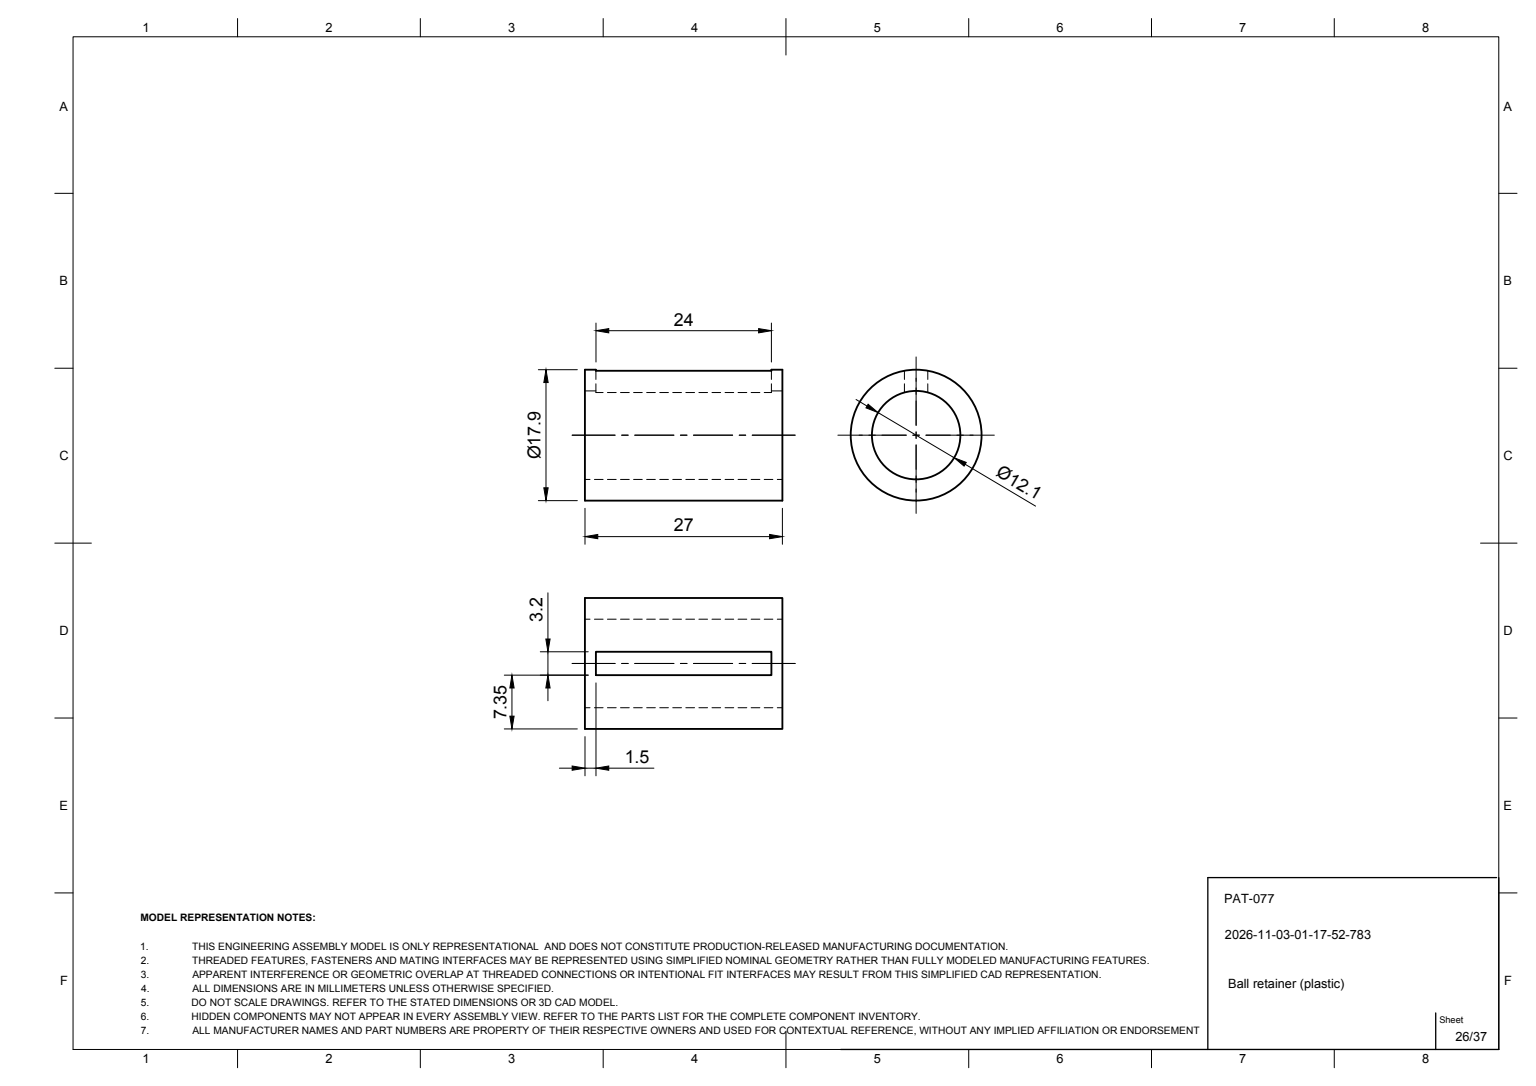
ISO-10303-21;
HEADER;
/* Generated by software containing ST-Developer
 * from STEP Tools, Inc. (www.steptools.com) 
 */

FILE_DESCRIPTION(
/* description */ ('Pallet stop with pneumatic fitting'),
/* implementation_level */ '2;1');

FILE_NAME(
/* name */ 'Ball retainer (plastic).step',
/* time_stamp */ '2026-10-27T10:51:41-07:00',
/* author */ (''),
/* organization */ (''),
/* preprocessor_version */ 'ST-DEVELOPER v20.2',
/* originating_system */ 'Autodesk Translation Framework v15.17.0.0',
/* authorisation */ '');

FILE_SCHEMA (('AUTOMOTIVE_DESIGN { 1 0 10303 214 3 1 1 }'));
ENDSEC;

DATA;
#10=MECHANICAL_DESIGN_GEOMETRIC_PRESENTATION_REPRESENTATION('',(#376),#10265);
#312=SHAPE_REPRESENTATION_RELATIONSHIP('SRR','None',#10426,#344);
#344=ADVANCED_BREP_SHAPE_REPRESENTATION('',(#408),#10250);
#376=STYLED_ITEM('',(#10648),#408);
#408=MANIFOLD_SOLID_BREP('Body1',#5064);
#511=FACE_BOUND('',#1322,.T.);
#512=FACE_BOUND('',#1324,.T.);
#513=FACE_BOUND('',#1326,.T.);
#514=FACE_BOUND('',#1328,.T.);
#643=PLANE('',#5785);
#644=PLANE('',#5788);
#645=PLANE('',#5789);
#646=PLANE('',#5792);
#647=PLANE('',#5793);
#648=PLANE('',#5798);
#911=FACE_OUTER_BOUND('',#1317,.T.);
#912=FACE_OUTER_BOUND('',#1318,.T.);
#913=FACE_OUTER_BOUND('',#1319,.T.);
#914=FACE_OUTER_BOUND('',#1320,.T.);
#915=FACE_OUTER_BOUND('',#1321,.T.);
#916=FACE_OUTER_BOUND('',#1323,.T.);
#917=FACE_OUTER_BOUND('',#1325,.T.);
#918=FACE_OUTER_BOUND('',#1327,.T.);
#1317=EDGE_LOOP('',(#4060,#4061,#4062,#4063));
#1318=EDGE_LOOP('',(#4064,#4065,#4066,#4067));
#1319=EDGE_LOOP('',(#4068,#4069,#4070,#4071));
#1320=EDGE_LOOP('',(#4072,#4073,#4074,#4075));
#1321=EDGE_LOOP('',(#4076));
#1322=EDGE_LOOP('',(#4077));
#1323=EDGE_LOOP('',(#4078,#4079,#4080,#4081));
#1324=EDGE_LOOP('',(#4082,#4083,#4084,#4085));
#1325=EDGE_LOOP('',(#4086));
#1326=EDGE_LOOP('',(#4087));
#1327=EDGE_LOOP('',(#4088,#4089,#4090,#4091));
#1328=EDGE_LOOP('',(#4092,#4093,#4094,#4095));
#1652=LINE('',#9434,#1987);
#1653=LINE('',#9437,#1988);
#1654=LINE('',#9440,#1989);
#1655=LINE('',#9442,#1990);
#1656=LINE('',#9443,#1991);
#1657=LINE('',#9449,#1992);
#1658=LINE('',#9451,#1993);
#1659=LINE('',#9452,#1994);
#1660=LINE('',#9461,#1995);
#1661=LINE('',#9466,#1996);
#1987=VECTOR('',#6961,1.);
#1988=VECTOR('',#6964,1.);
#1989=VECTOR('',#6967,1.);
#1990=VECTOR('',#6968,1.);
#1991=VECTOR('',#6969,1.);
#1992=VECTOR('',#6976,1.);
#1993=VECTOR('',#6979,1.);
#1994=VECTOR('',#6980,1.);
#1995=VECTOR('',#6991,0.895);
#1996=VECTOR('',#6998,0.605);
#2316=CIRCLE('',#5786,0.895);
#2317=CIRCLE('',#5787,0.605);
#2318=CIRCLE('',#5790,0.895);
#2319=CIRCLE('',#5791,0.605);
#2320=CIRCLE('',#5794,0.895);
#2321=CIRCLE('',#5795,0.605);
#2322=CIRCLE('',#5797,0.895);
#2323=CIRCLE('',#5799,0.605);
#2622=VERTEX_POINT('',#9430);
#2623=VERTEX_POINT('',#9431);
#2624=VERTEX_POINT('',#9433);
#2625=VERTEX_POINT('',#9435);
#2626=VERTEX_POINT('',#9439);
#2627=VERTEX_POINT('',#9441);
#2628=VERTEX_POINT('',#9445);
#2629=VERTEX_POINT('',#9447);
#2630=VERTEX_POINT('',#9454);
#2631=VERTEX_POINT('',#9456);
#2632=VERTEX_POINT('',#9459);
#2633=VERTEX_POINT('',#9463);
#3129=EDGE_CURVE('',#2622,#2623,#2316,.T.);
#3130=EDGE_CURVE('',#2624,#2622,#1652,.T.);
#3131=EDGE_CURVE('',#2625,#2624,#2317,.T.);
#3132=EDGE_CURVE('',#2623,#2625,#1653,.T.);
#3133=EDGE_CURVE('',#2623,#2626,#1654,.T.);
#3134=EDGE_CURVE('',#2627,#2625,#1655,.T.);
#3135=EDGE_CURVE('',#2627,#2626,#1656,.T.);
#3136=EDGE_CURVE('',#2626,#2628,#2318,.T.);
#3137=EDGE_CURVE('',#2629,#2627,#2319,.T.);
#3138=EDGE_CURVE('',#2628,#2629,#1657,.T.);
#3139=EDGE_CURVE('',#2628,#2622,#1658,.T.);
#3140=EDGE_CURVE('',#2624,#2629,#1659,.T.);
#3141=EDGE_CURVE('',#2630,#2630,#2320,.T.);
#3142=EDGE_CURVE('',#2631,#2631,#2321,.T.);
#3143=EDGE_CURVE('',#2632,#2632,#2322,.T.);
#3144=EDGE_CURVE('',#2632,#2630,#1660,.T.);
#3145=EDGE_CURVE('',#2633,#2633,#2323,.T.);
#3146=EDGE_CURVE('',#2633,#2631,#1661,.T.);
#4060=ORIENTED_EDGE('',*,*,#3129,.F.);
#4061=ORIENTED_EDGE('',*,*,#3130,.F.);
#4062=ORIENTED_EDGE('',*,*,#3131,.F.);
#4063=ORIENTED_EDGE('',*,*,#3132,.F.);
#4064=ORIENTED_EDGE('',*,*,#3133,.F.);
#4065=ORIENTED_EDGE('',*,*,#3132,.T.);
#4066=ORIENTED_EDGE('',*,*,#3134,.F.);
#4067=ORIENTED_EDGE('',*,*,#3135,.T.);
#4068=ORIENTED_EDGE('',*,*,#3136,.F.);
#4069=ORIENTED_EDGE('',*,*,#3135,.F.);
#4070=ORIENTED_EDGE('',*,*,#3137,.F.);
#4071=ORIENTED_EDGE('',*,*,#3138,.F.);
#4072=ORIENTED_EDGE('',*,*,#3139,.F.);
#4073=ORIENTED_EDGE('',*,*,#3138,.T.);
#4074=ORIENTED_EDGE('',*,*,#3140,.F.);
#4075=ORIENTED_EDGE('',*,*,#3130,.T.);
#4076=ORIENTED_EDGE('',*,*,#3141,.F.);
#4077=ORIENTED_EDGE('',*,*,#3142,.T.);
#4078=ORIENTED_EDGE('',*,*,#3143,.F.);
#4079=ORIENTED_EDGE('',*,*,#3144,.T.);
#4080=ORIENTED_EDGE('',*,*,#3141,.T.);
#4081=ORIENTED_EDGE('',*,*,#3144,.F.);
#4082=ORIENTED_EDGE('',*,*,#3136,.T.);
#4083=ORIENTED_EDGE('',*,*,#3139,.T.);
#4084=ORIENTED_EDGE('',*,*,#3129,.T.);
#4085=ORIENTED_EDGE('',*,*,#3133,.T.);
#4086=ORIENTED_EDGE('',*,*,#3143,.T.);
#4087=ORIENTED_EDGE('',*,*,#3145,.F.);
#4088=ORIENTED_EDGE('',*,*,#3145,.T.);
#4089=ORIENTED_EDGE('',*,*,#3146,.T.);
#4090=ORIENTED_EDGE('',*,*,#3142,.F.);
#4091=ORIENTED_EDGE('',*,*,#3146,.F.);
#4092=ORIENTED_EDGE('',*,*,#3137,.T.);
#4093=ORIENTED_EDGE('',*,*,#3134,.T.);
#4094=ORIENTED_EDGE('',*,*,#3131,.T.);
#4095=ORIENTED_EDGE('',*,*,#3140,.T.);
#4698=CYLINDRICAL_SURFACE('',#5796,0.895);
#4699=CYLINDRICAL_SURFACE('',#5800,0.605);
#4906=ADVANCED_FACE('',(#911),#643,.F.);
#4907=ADVANCED_FACE('',(#912),#644,.F.);
#4908=ADVANCED_FACE('',(#913),#645,.F.);
#4909=ADVANCED_FACE('',(#914),#646,.F.);
#4910=ADVANCED_FACE('',(#915,#511),#647,.T.);
#4911=ADVANCED_FACE('',(#916,#512),#4698,.T.);
#4912=ADVANCED_FACE('',(#917,#513),#648,.T.);
#4913=ADVANCED_FACE('',(#918,#514),#4699,.F.);
#5064=CLOSED_SHELL('',(#4906,#4907,#4908,#4909,#4910,#4911,#4912,#4913));
#5784=AXIS2_PLACEMENT_3D('',#9428,#6955,#6956);
#5785=AXIS2_PLACEMENT_3D('',#9429,#6957,#6958);
#5786=AXIS2_PLACEMENT_3D('',#9432,#6959,#6960);
#5787=AXIS2_PLACEMENT_3D('',#9436,#6962,#6963);
#5788=AXIS2_PLACEMENT_3D('',#9438,#6965,#6966);
#5789=AXIS2_PLACEMENT_3D('',#9444,#6970,#6971);
#5790=AXIS2_PLACEMENT_3D('',#9446,#6972,#6973);
#5791=AXIS2_PLACEMENT_3D('',#9448,#6974,#6975);
#5792=AXIS2_PLACEMENT_3D('',#9450,#6977,#6978);
#5793=AXIS2_PLACEMENT_3D('',#9453,#6981,#6982);
#5794=AXIS2_PLACEMENT_3D('',#9455,#6983,#6984);
#5795=AXIS2_PLACEMENT_3D('',#9457,#6985,#6986);
#5796=AXIS2_PLACEMENT_3D('',#9458,#6987,#6988);
#5797=AXIS2_PLACEMENT_3D('',#9460,#6989,#6990);
#5798=AXIS2_PLACEMENT_3D('',#9462,#6992,#6993);
#5799=AXIS2_PLACEMENT_3D('',#9464,#6994,#6995);
#5800=AXIS2_PLACEMENT_3D('',#9465,#6996,#6997);
#6955=DIRECTION('axis',(0.,0.,1.));
#6956=DIRECTION('refdir',(1.,0.,0.));
#6957=DIRECTION('center_axis',(0.,1.,0.));
#6958=DIRECTION('ref_axis',(0.,0.,1.));
#6959=DIRECTION('center_axis',(0.,1.,0.));
#6960=DIRECTION('ref_axis',(1.,0.,0.));
#6961=DIRECTION('',(1.,0.,0.));
#6962=DIRECTION('center_axis',(0.,-1.,0.));
#6963=DIRECTION('ref_axis',(1.,0.,0.));
#6964=DIRECTION('',(-1.,0.,0.));
#6965=DIRECTION('center_axis',(0.,0.,-1.));
#6966=DIRECTION('ref_axis',(-1.,0.,0.));
#6967=DIRECTION('',(0.,-1.,0.));
#6968=DIRECTION('',(0.,1.,0.));
#6969=DIRECTION('',(1.,0.,0.));
#6970=DIRECTION('center_axis',(0.,-1.,0.));
#6971=DIRECTION('ref_axis',(0.,0.,-1.));
#6972=DIRECTION('center_axis',(0.,-1.,0.));
#6973=DIRECTION('ref_axis',(1.,0.,0.));
#6974=DIRECTION('center_axis',(0.,1.,0.));
#6975=DIRECTION('ref_axis',(1.,0.,0.));
#6976=DIRECTION('',(-1.,0.,0.));
#6977=DIRECTION('center_axis',(0.,0.,1.));
#6978=DIRECTION('ref_axis',(1.,0.,0.));
#6979=DIRECTION('',(0.,1.,0.));
#6980=DIRECTION('',(0.,-1.,0.));
#6981=DIRECTION('center_axis',(0.,1.,0.));
#6982=DIRECTION('ref_axis',(0.,0.,1.));
#6983=DIRECTION('center_axis',(0.,-1.,0.));
#6984=DIRECTION('ref_axis',(1.,0.,0.));
#6985=DIRECTION('center_axis',(0.,-1.,0.));
#6986=DIRECTION('ref_axis',(1.,0.,0.));
#6987=DIRECTION('center_axis',(0.,-1.,0.));
#6988=DIRECTION('ref_axis',(1.,0.,0.));
#6989=DIRECTION('center_axis',(0.,-1.,0.));
#6990=DIRECTION('ref_axis',(1.,0.,0.));
#6991=DIRECTION('',(0.,1.,0.));
#6992=DIRECTION('center_axis',(0.,-1.,0.));
#6993=DIRECTION('ref_axis',(0.,0.,-1.));
#6994=DIRECTION('center_axis',(0.,-1.,0.));
#6995=DIRECTION('ref_axis',(1.,0.,0.));
#6996=DIRECTION('center_axis',(0.,-1.,0.));
#6997=DIRECTION('ref_axis',(1.,0.,0.));
#6998=DIRECTION('',(0.,1.,0.));
#9428=CARTESIAN_POINT('',(0.,0.,0.));
#9429=CARTESIAN_POINT('Origin',(0.75,1.2,0.));
#9430=CARTESIAN_POINT('',(0.880582193778639,1.2,0.16));
#9431=CARTESIAN_POINT('',(0.880582193778639,1.2,-0.16));
#9432=CARTESIAN_POINT('Origin',(0.,1.2,0.));
#9433=CARTESIAN_POINT('',(0.583459510163302,1.2,0.16));
#9434=CARTESIAN_POINT('',(0.57,1.2,0.16));
#9435=CARTESIAN_POINT('',(0.583459510163302,1.2,-0.16));
#9436=CARTESIAN_POINT('Origin',(0.,1.2,0.));
#9437=CARTESIAN_POINT('',(0.93,1.2,-0.16));
#9438=CARTESIAN_POINT('Origin',(0.93,0.,-0.16));
#9439=CARTESIAN_POINT('',(0.880582193778639,-1.2,-0.16));
#9440=CARTESIAN_POINT('',(0.880582193778639,0.,-0.16));
#9441=CARTESIAN_POINT('',(0.583459510163302,-1.2,-0.16));
#9442=CARTESIAN_POINT('',(0.583459510163302,0.,-0.16));
#9443=CARTESIAN_POINT('',(0.93,-1.2,-0.16));
#9444=CARTESIAN_POINT('Origin',(0.75,-1.2,0.));
#9445=CARTESIAN_POINT('',(0.880582193778639,-1.2,0.16));
#9446=CARTESIAN_POINT('Origin',(0.,-1.2,0.));
#9447=CARTESIAN_POINT('',(0.583459510163302,-1.2,0.16));
#9448=CARTESIAN_POINT('Origin',(0.,-1.2,0.));
#9449=CARTESIAN_POINT('',(0.57,-1.2,0.16));
#9450=CARTESIAN_POINT('Origin',(0.57,0.,0.16));
#9451=CARTESIAN_POINT('',(0.880582193778639,0.,0.16));
#9452=CARTESIAN_POINT('',(0.583459510163302,0.,0.16));
#9453=CARTESIAN_POINT('Origin',(0.895,1.35,0.));
#9454=CARTESIAN_POINT('',(-0.895,1.35,-1.09605888523688E-16));
#9455=CARTESIAN_POINT('Origin',(0.,1.35,0.));
#9456=CARTESIAN_POINT('',(-0.605,1.35,-7.40911313484149E-17));
#9457=CARTESIAN_POINT('Origin',(0.,1.35,0.));
#9458=CARTESIAN_POINT('Origin',(0.,0.,0.));
#9459=CARTESIAN_POINT('',(-0.895,-1.35,-1.09605888523688E-16));
#9460=CARTESIAN_POINT('Origin',(0.,-1.35,0.));
#9461=CARTESIAN_POINT('',(-0.895,0.,-1.09605888523688E-16));
#9462=CARTESIAN_POINT('Origin',(0.605,-1.35,0.));
#9463=CARTESIAN_POINT('',(-0.605,-1.35,-7.40911313484149E-17));
#9464=CARTESIAN_POINT('Origin',(0.,-1.35,0.));
#9465=CARTESIAN_POINT('Origin',(0.,0.,0.));
#9466=CARTESIAN_POINT('',(-0.605,0.,-7.40911313484149E-17));
#10212=UNCERTAINTY_MEASURE_WITH_UNIT(LENGTH_MEASURE(0.001),#10266,
'DISTANCE_ACCURACY_VALUE',
'Maximum model space distance between geometric entities at asserted c
onnectivities');
#10227=UNCERTAINTY_MEASURE_WITH_UNIT(LENGTH_MEASURE(0.001),#10266,
'DISTANCE_ACCURACY_VALUE',
'Maximum model space distance between geometric entities at asserted c
onnectivities');
#10250=(
GEOMETRIC_REPRESENTATION_CONTEXT(3)
GLOBAL_UNCERTAINTY_ASSIGNED_CONTEXT((#10212))
GLOBAL_UNIT_ASSIGNED_CONTEXT((#10266,#10268,#10269))
REPRESENTATION_CONTEXT('','3D')
);
#10265=(
GEOMETRIC_REPRESENTATION_CONTEXT(3)
GLOBAL_UNCERTAINTY_ASSIGNED_CONTEXT((#10227))
GLOBAL_UNIT_ASSIGNED_CONTEXT((#10266,#10268,#10269))
REPRESENTATION_CONTEXT('','3D')
);
#10266=(
LENGTH_UNIT()
NAMED_UNIT(*)
SI_UNIT(.CENTI.,.METRE.)
);
#10268=(
NAMED_UNIT(*)
PLANE_ANGLE_UNIT()
SI_UNIT($,.RADIAN.)
);
#10269=(
NAMED_UNIT(*)
SI_UNIT($,.STERADIAN.)
SOLID_ANGLE_UNIT()
);
#10292=SHAPE_DEFINITION_REPRESENTATION(#10329,#10426);
#10329=PRODUCT_DEFINITION_SHAPE('',$,#10464);
#10426=SHAPE_REPRESENTATION('',(#5784),#10250);
#10441=PRODUCT_DEFINITION_CONTEXT('part definition',#10554,'design');
#10464=PRODUCT_DEFINITION('Ball retainer (plastic)',
'Ball retainer (plastic)',#10501,#10441);
#10501=PRODUCT_DEFINITION_FORMATION('',$,#10578);
#10554=APPLICATION_CONTEXT(
'Core Data for Automotive Mechanical Design Process');
#10555=PRODUCT_CONTEXT('part definition',#10554,'mechanical');
#10578=PRODUCT('Ball retainer (plastic)','Ball retainer (plastic)',
'Ball retainer (plastic)',(#10555));
#10642=COLOUR_RGB('Sky Blue',0.24,0.69,0.87);
#10643=FILL_AREA_STYLE_COLOUR('',#10642);
#10644=FILL_AREA_STYLE('',(#10643));
#10645=SURFACE_STYLE_FILL_AREA(#10644);
#10646=SURFACE_SIDE_STYLE('',(#10645));
#10647=SURFACE_STYLE_USAGE(.BOTH.,#10646);
#10648=PRESENTATION_STYLE_ASSIGNMENT((#10647));
ENDSEC;
END-ISO-10303-21;
